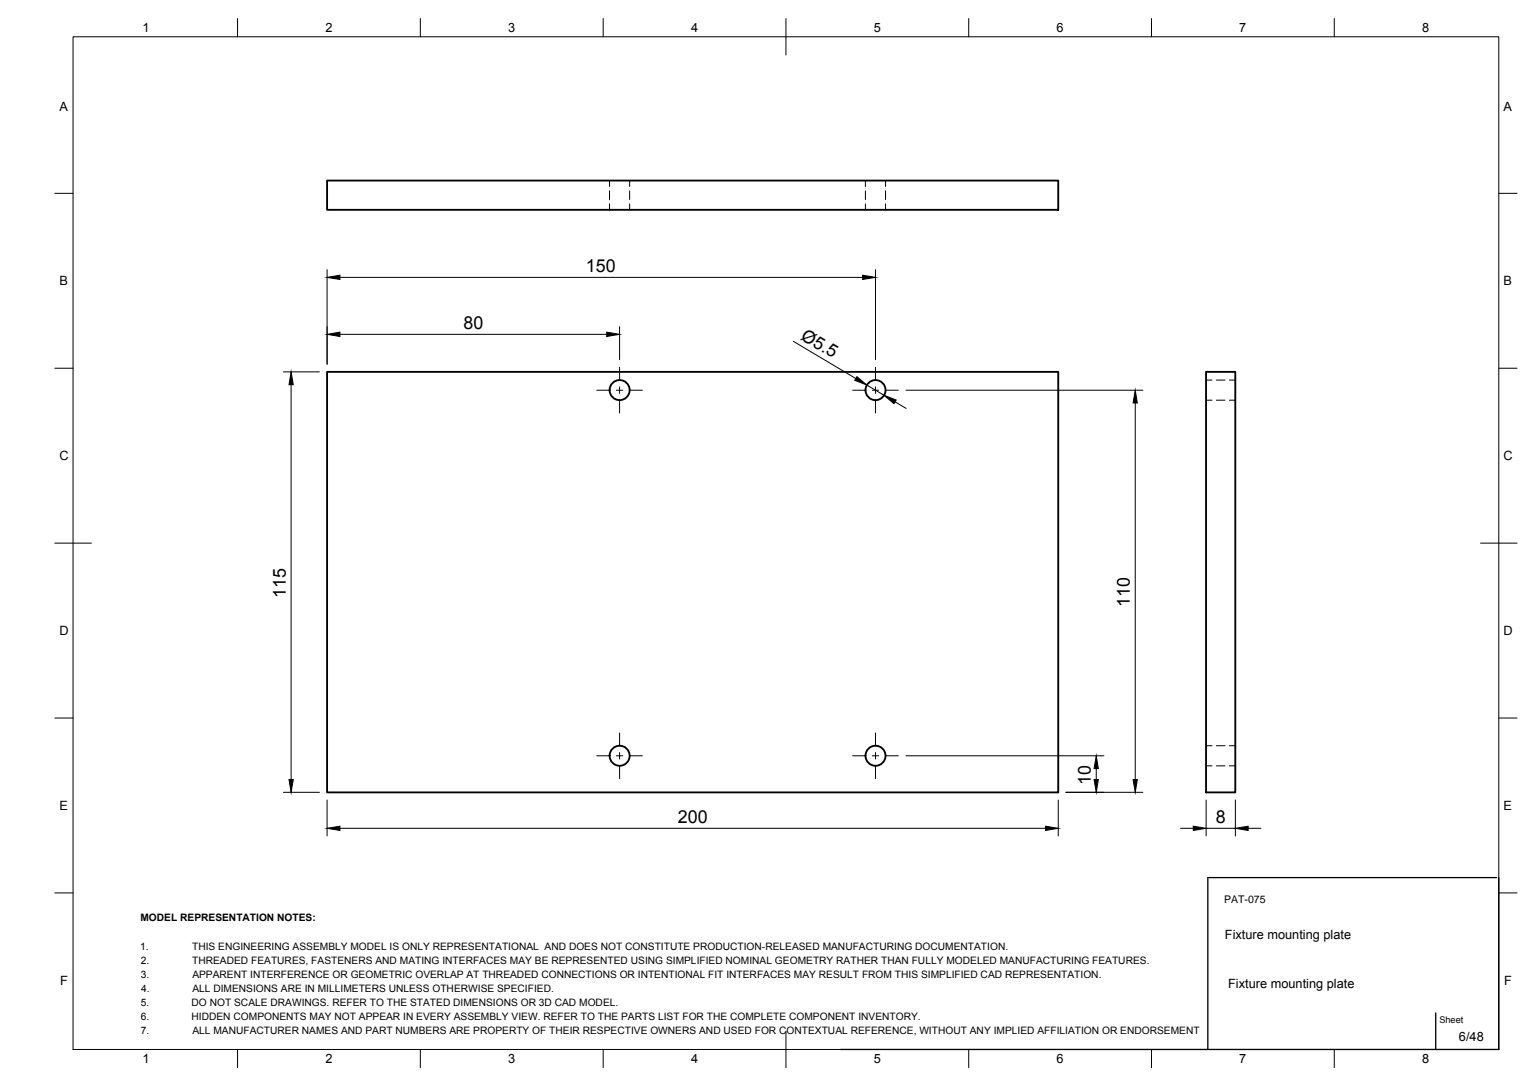
ISO-10303-21;
HEADER;
/* Generated by software containing ST-Developer
 * from STEP Tools, Inc. (www.steptools.com) 
 */

FILE_DESCRIPTION(
/* description */ ('Over-Centre Plunger Toggle Clamp on Slotted Fixture Frame'),
/* implementation_level */ '2;1');

FILE_NAME(
/* name */ 
'Fixture mounting plate.step',
/* time_stamp */ '2026-10-28T03:23:24-07:00',
/* author */ (''),
/* organization */ (''),
/* preprocessor_version */ 'ST-DEVELOPER v20.2',
/* originating_system */ 'Autodesk Translation Framework v15.17.0.0',
/* authorisation */ '');

FILE_SCHEMA (('AUTOMOTIVE_DESIGN { 1 0 10303 214 3 1 1 }'));
ENDSEC;

DATA;
#10=MECHANICAL_DESIGN_GEOMETRIC_PRESENTATION_REPRESENTATION('',(#514),#15212);
#430=SHAPE_REPRESENTATION_RELATIONSHIP('SRR','None',#15404,#472);
#472=ADVANCED_BREP_SHAPE_REPRESENTATION('',(#565),#15166);
#514=STYLED_ITEM('',(#15712),#565);
#565=MANIFOLD_SOLID_BREP('Body1',#8246);
#635=FACE_BOUND('',#1624,.T.);
#636=FACE_BOUND('',#1625,.T.);
#637=FACE_BOUND('',#1626,.T.);
#638=FACE_BOUND('',#1627,.T.);
#639=FACE_BOUND('',#1629,.T.);
#640=FACE_BOUND('',#1630,.T.);
#641=FACE_BOUND('',#1631,.T.);
#642=FACE_BOUND('',#1632,.T.);
#789=PLANE('',#8821);
#790=PLANE('',#8822);
#791=PLANE('',#8823);
#792=PLANE('',#8824);
#793=PLANE('',#8825);
#794=PLANE('',#8826);
#1105=FACE_OUTER_BOUND('',#1615,.T.);
#1106=FACE_OUTER_BOUND('',#1616,.T.);
#1107=FACE_OUTER_BOUND('',#1617,.T.);
#1108=FACE_OUTER_BOUND('',#1618,.T.);
#1109=FACE_OUTER_BOUND('',#1619,.T.);
#1110=FACE_OUTER_BOUND('',#1620,.T.);
#1111=FACE_OUTER_BOUND('',#1621,.T.);
#1112=FACE_OUTER_BOUND('',#1622,.T.);
#1113=FACE_OUTER_BOUND('',#1623,.T.);
#1114=FACE_OUTER_BOUND('',#1628,.T.);
#1615=EDGE_LOOP('',(#5665,#5666,#5667,#5668));
#1616=EDGE_LOOP('',(#5669,#5670,#5671,#5672));
#1617=EDGE_LOOP('',(#5673,#5674,#5675,#5676));
#1618=EDGE_LOOP('',(#5677,#5678,#5679,#5680));
#1619=EDGE_LOOP('',(#5681,#5682,#5683,#5684));
#1620=EDGE_LOOP('',(#5685,#5686,#5687,#5688));
#1621=EDGE_LOOP('',(#5689,#5690,#5691,#5692));
#1622=EDGE_LOOP('',(#5693,#5694,#5695,#5696));
#1623=EDGE_LOOP('',(#5697,#5698,#5699,#5700));
#1624=EDGE_LOOP('',(#5701));
#1625=EDGE_LOOP('',(#5702));
#1626=EDGE_LOOP('',(#5703));
#1627=EDGE_LOOP('',(#5704));
#1628=EDGE_LOOP('',(#5705,#5706,#5707,#5708));
#1629=EDGE_LOOP('',(#5709));
#1630=EDGE_LOOP('',(#5710));
#1631=EDGE_LOOP('',(#5711));
#1632=EDGE_LOOP('',(#5712));
#2255=LINE('',#12472,#2885);
#2256=LINE('',#12478,#2886);
#2257=LINE('',#12484,#2887);
#2258=LINE('',#12490,#2888);
#2259=LINE('',#12495,#2889);
#2260=LINE('',#12497,#2890);
#2261=LINE('',#12499,#2891);
#2262=LINE('',#12500,#2892);
#2263=LINE('',#12503,#2893);
#2264=LINE('',#12505,#2894);
#2265=LINE('',#12506,#2895);
#2266=LINE('',#12509,#2896);
#2267=LINE('',#12511,#2897);
#2268=LINE('',#12512,#2898);
#2269=LINE('',#12514,#2899);
#2270=LINE('',#12515,#2900);
#2885=VECTOR('',#9874,0.275);
#2886=VECTOR('',#9881,0.275);
#2887=VECTOR('',#9888,0.275);
#2888=VECTOR('',#9895,0.275);
#2889=VECTOR('',#9900,1.);
#2890=VECTOR('',#9901,1.);
#2891=VECTOR('',#9902,1.);
#2892=VECTOR('',#9903,1.);
#2893=VECTOR('',#9906,1.);
#2894=VECTOR('',#9907,1.);
#2895=VECTOR('',#9908,1.);
#2896=VECTOR('',#9911,1.);
#2897=VECTOR('',#9912,1.);
#2898=VECTOR('',#9913,1.);
#2899=VECTOR('',#9916,1.);
#2900=VECTOR('',#9917,1.);
#3515=CIRCLE('',#8810,0.275);
#3516=CIRCLE('',#8811,0.275);
#3517=CIRCLE('',#8813,0.275);
#3518=CIRCLE('',#8814,0.275);
#3519=CIRCLE('',#8816,0.275);
#3520=CIRCLE('',#8817,0.275);
#3521=CIRCLE('',#8819,0.275);
#3522=CIRCLE('',#8820,0.275);
#3891=VERTEX_POINT('',#12469);
#3892=VERTEX_POINT('',#12471);
#3893=VERTEX_POINT('',#12475);
#3894=VERTEX_POINT('',#12477);
#3895=VERTEX_POINT('',#12481);
#3896=VERTEX_POINT('',#12483);
#3897=VERTEX_POINT('',#12487);
#3898=VERTEX_POINT('',#12489);
#3899=VERTEX_POINT('',#12493);
#3900=VERTEX_POINT('',#12494);
#3901=VERTEX_POINT('',#12496);
#3902=VERTEX_POINT('',#12498);
#3903=VERTEX_POINT('',#12502);
#3904=VERTEX_POINT('',#12504);
#3905=VERTEX_POINT('',#12508);
#3906=VERTEX_POINT('',#12510);
#4593=EDGE_CURVE('',#3891,#3891,#3515,.T.);
#4594=EDGE_CURVE('',#3891,#3892,#2255,.T.);
#4595=EDGE_CURVE('',#3892,#3892,#3516,.T.);
#4596=EDGE_CURVE('',#3893,#3893,#3517,.T.);
#4597=EDGE_CURVE('',#3893,#3894,#2256,.T.);
#4598=EDGE_CURVE('',#3894,#3894,#3518,.T.);
#4599=EDGE_CURVE('',#3895,#3895,#3519,.T.);
#4600=EDGE_CURVE('',#3895,#3896,#2257,.T.);
#4601=EDGE_CURVE('',#3896,#3896,#3520,.T.);
#4602=EDGE_CURVE('',#3897,#3897,#3521,.T.);
#4603=EDGE_CURVE('',#3897,#3898,#2258,.T.);
#4604=EDGE_CURVE('',#3898,#3898,#3522,.T.);
#4605=EDGE_CURVE('',#3899,#3900,#2259,.T.);
#4606=EDGE_CURVE('',#3900,#3901,#2260,.T.);
#4607=EDGE_CURVE('',#3902,#3901,#2261,.T.);
#4608=EDGE_CURVE('',#3899,#3902,#2262,.T.);
#4609=EDGE_CURVE('',#3903,#3899,#2263,.T.);
#4610=EDGE_CURVE('',#3904,#3902,#2264,.T.);
#4611=EDGE_CURVE('',#3903,#3904,#2265,.T.);
#4612=EDGE_CURVE('',#3905,#3903,#2266,.T.);
#4613=EDGE_CURVE('',#3906,#3904,#2267,.T.);
#4614=EDGE_CURVE('',#3905,#3906,#2268,.T.);
#4615=EDGE_CURVE('',#3900,#3905,#2269,.T.);
#4616=EDGE_CURVE('',#3901,#3906,#2270,.T.);
#5665=ORIENTED_EDGE('',*,*,#4593,.F.);
#5666=ORIENTED_EDGE('',*,*,#4594,.T.);
#5667=ORIENTED_EDGE('',*,*,#4595,.F.);
#5668=ORIENTED_EDGE('',*,*,#4594,.F.);
#5669=ORIENTED_EDGE('',*,*,#4596,.F.);
#5670=ORIENTED_EDGE('',*,*,#4597,.T.);
#5671=ORIENTED_EDGE('',*,*,#4598,.F.);
#5672=ORIENTED_EDGE('',*,*,#4597,.F.);
#5673=ORIENTED_EDGE('',*,*,#4599,.F.);
#5674=ORIENTED_EDGE('',*,*,#4600,.T.);
#5675=ORIENTED_EDGE('',*,*,#4601,.F.);
#5676=ORIENTED_EDGE('',*,*,#4600,.F.);
#5677=ORIENTED_EDGE('',*,*,#4602,.F.);
#5678=ORIENTED_EDGE('',*,*,#4603,.T.);
#5679=ORIENTED_EDGE('',*,*,#4604,.F.);
#5680=ORIENTED_EDGE('',*,*,#4603,.F.);
#5681=ORIENTED_EDGE('',*,*,#4605,.T.);
#5682=ORIENTED_EDGE('',*,*,#4606,.T.);
#5683=ORIENTED_EDGE('',*,*,#4607,.F.);
#5684=ORIENTED_EDGE('',*,*,#4608,.F.);
#5685=ORIENTED_EDGE('',*,*,#4609,.T.);
#5686=ORIENTED_EDGE('',*,*,#4608,.T.);
#5687=ORIENTED_EDGE('',*,*,#4610,.F.);
#5688=ORIENTED_EDGE('',*,*,#4611,.F.);
#5689=ORIENTED_EDGE('',*,*,#4612,.T.);
#5690=ORIENTED_EDGE('',*,*,#4611,.T.);
#5691=ORIENTED_EDGE('',*,*,#4613,.F.);
#5692=ORIENTED_EDGE('',*,*,#4614,.F.);
#5693=ORIENTED_EDGE('',*,*,#4615,.T.);
#5694=ORIENTED_EDGE('',*,*,#4614,.T.);
#5695=ORIENTED_EDGE('',*,*,#4616,.F.);
#5696=ORIENTED_EDGE('',*,*,#4606,.F.);
#5697=ORIENTED_EDGE('',*,*,#4616,.T.);
#5698=ORIENTED_EDGE('',*,*,#4613,.T.);
#5699=ORIENTED_EDGE('',*,*,#4610,.T.);
#5700=ORIENTED_EDGE('',*,*,#4607,.T.);
#5701=ORIENTED_EDGE('',*,*,#4595,.T.);
#5702=ORIENTED_EDGE('',*,*,#4598,.T.);
#5703=ORIENTED_EDGE('',*,*,#4601,.T.);
#5704=ORIENTED_EDGE('',*,*,#4604,.T.);
#5705=ORIENTED_EDGE('',*,*,#4615,.F.);
#5706=ORIENTED_EDGE('',*,*,#4605,.F.);
#5707=ORIENTED_EDGE('',*,*,#4609,.F.);
#5708=ORIENTED_EDGE('',*,*,#4612,.F.);
#5709=ORIENTED_EDGE('',*,*,#4593,.T.);
#5710=ORIENTED_EDGE('',*,*,#4596,.T.);
#5711=ORIENTED_EDGE('',*,*,#4599,.T.);
#5712=ORIENTED_EDGE('',*,*,#4602,.T.);
#7629=CYLINDRICAL_SURFACE('',#8809,0.275);
#7630=CYLINDRICAL_SURFACE('',#8812,0.275);
#7631=CYLINDRICAL_SURFACE('',#8815,0.275);
#7632=CYLINDRICAL_SURFACE('',#8818,0.275);
#7777=ADVANCED_FACE('',(#1105),#7629,.F.);
#7778=ADVANCED_FACE('',(#1106),#7630,.F.);
#7779=ADVANCED_FACE('',(#1107),#7631,.F.);
#7780=ADVANCED_FACE('',(#1108),#7632,.F.);
#7781=ADVANCED_FACE('',(#1109),#789,.T.);
#7782=ADVANCED_FACE('',(#1110),#790,.T.);
#7783=ADVANCED_FACE('',(#1111),#791,.T.);
#7784=ADVANCED_FACE('',(#1112),#792,.T.);
#7785=ADVANCED_FACE('',(#1113,#635,#636,#637,#638),#793,.T.);
#7786=ADVANCED_FACE('',(#1114,#639,#640,#641,#642),#794,.F.);
#8246=CLOSED_SHELL('',(#7777,#7778,#7779,#7780,#7781,#7782,#7783,#7784,
#7785,#7786));
#8808=AXIS2_PLACEMENT_3D('',#12467,#9868,#9869);
#8809=AXIS2_PLACEMENT_3D('',#12468,#9870,#9871);
#8810=AXIS2_PLACEMENT_3D('',#12470,#9872,#9873);
#8811=AXIS2_PLACEMENT_3D('',#12473,#9875,#9876);
#8812=AXIS2_PLACEMENT_3D('',#12474,#9877,#9878);
#8813=AXIS2_PLACEMENT_3D('',#12476,#9879,#9880);
#8814=AXIS2_PLACEMENT_3D('',#12479,#9882,#9883);
#8815=AXIS2_PLACEMENT_3D('',#12480,#9884,#9885);
#8816=AXIS2_PLACEMENT_3D('',#12482,#9886,#9887);
#8817=AXIS2_PLACEMENT_3D('',#12485,#9889,#9890);
#8818=AXIS2_PLACEMENT_3D('',#12486,#9891,#9892);
#8819=AXIS2_PLACEMENT_3D('',#12488,#9893,#9894);
#8820=AXIS2_PLACEMENT_3D('',#12491,#9896,#9897);
#8821=AXIS2_PLACEMENT_3D('',#12492,#9898,#9899);
#8822=AXIS2_PLACEMENT_3D('',#12501,#9904,#9905);
#8823=AXIS2_PLACEMENT_3D('',#12507,#9909,#9910);
#8824=AXIS2_PLACEMENT_3D('',#12513,#9914,#9915);
#8825=AXIS2_PLACEMENT_3D('',#12516,#9918,#9919);
#8826=AXIS2_PLACEMENT_3D('',#12517,#9920,#9921);
#9868=DIRECTION('axis',(0.,0.,1.));
#9869=DIRECTION('refdir',(1.,0.,0.));
#9870=DIRECTION('center_axis',(0.,0.,1.));
#9871=DIRECTION('ref_axis',(1.,0.,0.));
#9872=DIRECTION('center_axis',(0.,0.,1.));
#9873=DIRECTION('ref_axis',(1.,0.,0.));
#9874=DIRECTION('',(0.,0.,1.));
#9875=DIRECTION('center_axis',(0.,0.,-1.));
#9876=DIRECTION('ref_axis',(1.,0.,0.));
#9877=DIRECTION('center_axis',(0.,0.,1.));
#9878=DIRECTION('ref_axis',(1.,0.,0.));
#9879=DIRECTION('center_axis',(0.,0.,1.));
#9880=DIRECTION('ref_axis',(1.,0.,0.));
#9881=DIRECTION('',(0.,0.,1.));
#9882=DIRECTION('center_axis',(0.,0.,-1.));
#9883=DIRECTION('ref_axis',(1.,0.,0.));
#9884=DIRECTION('center_axis',(0.,0.,1.));
#9885=DIRECTION('ref_axis',(1.,0.,0.));
#9886=DIRECTION('center_axis',(0.,0.,1.));
#9887=DIRECTION('ref_axis',(1.,0.,0.));
#9888=DIRECTION('',(0.,0.,1.));
#9889=DIRECTION('center_axis',(0.,0.,-1.));
#9890=DIRECTION('ref_axis',(1.,0.,0.));
#9891=DIRECTION('center_axis',(0.,0.,1.));
#9892=DIRECTION('ref_axis',(1.,0.,0.));
#9893=DIRECTION('center_axis',(0.,0.,1.));
#9894=DIRECTION('ref_axis',(1.,0.,0.));
#9895=DIRECTION('',(0.,0.,1.));
#9896=DIRECTION('center_axis',(0.,0.,-1.));
#9897=DIRECTION('ref_axis',(1.,0.,0.));
#9898=DIRECTION('center_axis',(0.,1.,0.));
#9899=DIRECTION('ref_axis',(-1.,0.,0.));
#9900=DIRECTION('',(-1.,0.,0.));
#9901=DIRECTION('',(0.,0.,1.));
#9902=DIRECTION('',(-1.,0.,0.));
#9903=DIRECTION('',(0.,0.,1.));
#9904=DIRECTION('center_axis',(1.,0.,0.));
#9905=DIRECTION('ref_axis',(0.,1.,0.));
#9906=DIRECTION('',(0.,1.,0.));
#9907=DIRECTION('',(0.,1.,0.));
#9908=DIRECTION('',(0.,0.,1.));
#9909=DIRECTION('center_axis',(0.,-1.,0.));
#9910=DIRECTION('ref_axis',(1.,0.,0.));
#9911=DIRECTION('',(1.,0.,0.));
#9912=DIRECTION('',(1.,0.,0.));
#9913=DIRECTION('',(0.,0.,1.));
#9914=DIRECTION('center_axis',(-1.,0.,0.));
#9915=DIRECTION('ref_axis',(0.,-1.,0.));
#9916=DIRECTION('',(0.,-1.,0.));
#9917=DIRECTION('',(0.,-1.,0.));
#9918=DIRECTION('center_axis',(0.,0.,1.));
#9919=DIRECTION('ref_axis',(1.,0.,0.));
#9920=DIRECTION('center_axis',(0.,0.,1.));
#9921=DIRECTION('ref_axis',(1.,0.,0.));
#12467=CARTESIAN_POINT('',(0.,0.,0.));
#12468=CARTESIAN_POINT('Origin',(2.5,4.,-2.9));
#12469=CARTESIAN_POINT('',(2.225,4.,-2.8));
#12470=CARTESIAN_POINT('Origin',(2.5,4.,-2.8));
#12471=CARTESIAN_POINT('',(2.225,4.,-2.));
#12472=CARTESIAN_POINT('',(2.225,4.,-2.9));
#12473=CARTESIAN_POINT('Origin',(2.5,4.,-2.));
#12474=CARTESIAN_POINT('Origin',(-4.5,4.,-2.9));
#12475=CARTESIAN_POINT('',(-4.775,4.,-2.8));
#12476=CARTESIAN_POINT('Origin',(-4.5,4.,-2.8));
#12477=CARTESIAN_POINT('',(-4.775,4.,-2.));
#12478=CARTESIAN_POINT('',(-4.775,4.,-2.9));
#12479=CARTESIAN_POINT('Origin',(-4.5,4.,-2.));
#12480=CARTESIAN_POINT('Origin',(2.5,-6.,-2.9));
#12481=CARTESIAN_POINT('',(2.225,-6.,-2.8));
#12482=CARTESIAN_POINT('Origin',(2.5,-6.,-2.8));
#12483=CARTESIAN_POINT('',(2.225,-6.,-2.));
#12484=CARTESIAN_POINT('',(2.225,-6.,-2.9));
#12485=CARTESIAN_POINT('Origin',(2.5,-6.,-2.));
#12486=CARTESIAN_POINT('Origin',(-4.5,-6.,-2.9));
#12487=CARTESIAN_POINT('',(-4.775,-6.,-2.8));
#12488=CARTESIAN_POINT('Origin',(-4.5,-6.,-2.8));
#12489=CARTESIAN_POINT('',(-4.775,-6.,-2.));
#12490=CARTESIAN_POINT('',(-4.775,-6.,-2.9));
#12491=CARTESIAN_POINT('Origin',(-4.5,-6.,-2.));
#12492=CARTESIAN_POINT('Origin',(10.5,4.5,-2.8));
#12493=CARTESIAN_POINT('',(10.5,4.5,-2.8));
#12494=CARTESIAN_POINT('',(-9.5,4.5,-2.8));
#12495=CARTESIAN_POINT('',(10.5,4.5,-2.8));
#12496=CARTESIAN_POINT('',(-9.5,4.5,-2.));
#12497=CARTESIAN_POINT('',(-9.5,4.5,-2.8));
#12498=CARTESIAN_POINT('',(10.5,4.5,-2.));
#12499=CARTESIAN_POINT('',(10.5,4.5,-2.));
#12500=CARTESIAN_POINT('',(10.5,4.5,-2.8));
#12501=CARTESIAN_POINT('Origin',(10.5,-7.,-2.8));
#12502=CARTESIAN_POINT('',(10.5,-7.,-2.8));
#12503=CARTESIAN_POINT('',(10.5,-7.,-2.8));
#12504=CARTESIAN_POINT('',(10.5,-7.,-2.));
#12505=CARTESIAN_POINT('',(10.5,-7.,-2.));
#12506=CARTESIAN_POINT('',(10.5,-7.,-2.8));
#12507=CARTESIAN_POINT('Origin',(-9.5,-7.,-2.8));
#12508=CARTESIAN_POINT('',(-9.5,-7.,-2.8));
#12509=CARTESIAN_POINT('',(-9.5,-7.,-2.8));
#12510=CARTESIAN_POINT('',(-9.5,-7.,-2.));
#12511=CARTESIAN_POINT('',(-9.5,-7.,-2.));
#12512=CARTESIAN_POINT('',(-9.5,-7.,-2.8));
#12513=CARTESIAN_POINT('Origin',(-9.5,4.5,-2.8));
#12514=CARTESIAN_POINT('',(-9.5,4.5,-2.8));
#12515=CARTESIAN_POINT('',(-9.5,4.5,-2.));
#12516=CARTESIAN_POINT('Origin',(0.5,-1.25,-2.));
#12517=CARTESIAN_POINT('Origin',(0.5,-1.25,-2.8));
#15116=UNCERTAINTY_MEASURE_WITH_UNIT(LENGTH_MEASURE(0.001),#15213,
'DISTANCE_ACCURACY_VALUE',
'Maximum model space distance between geometric entities at asserted c
onnectivities');
#15162=UNCERTAINTY_MEASURE_WITH_UNIT(LENGTH_MEASURE(0.001),#15213,
'DISTANCE_ACCURACY_VALUE',
'Maximum model space distance between geometric entities at asserted c
onnectivities');
#15166=(
GEOMETRIC_REPRESENTATION_CONTEXT(3)
GLOBAL_UNCERTAINTY_ASSIGNED_CONTEXT((#15116))
GLOBAL_UNIT_ASSIGNED_CONTEXT((#15213,#15215,#15216))
REPRESENTATION_CONTEXT('','3D')
);
#15212=(
GEOMETRIC_REPRESENTATION_CONTEXT(3)
GLOBAL_UNCERTAINTY_ASSIGNED_CONTEXT((#15162))
GLOBAL_UNIT_ASSIGNED_CONTEXT((#15213,#15215,#15216))
REPRESENTATION_CONTEXT('','3D')
);
#15213=(
LENGTH_UNIT()
NAMED_UNIT(*)
SI_UNIT(.CENTI.,.METRE.)
);
#15215=(
NAMED_UNIT(*)
PLANE_ANGLE_UNIT()
SI_UNIT($,.RADIAN.)
);
#15216=(
NAMED_UNIT(*)
SI_UNIT($,.STERADIAN.)
SOLID_ANGLE_UNIT()
);
#15220=SHAPE_DEFINITION_REPRESENTATION(#15269,#15404);
#15269=PRODUCT_DEFINITION_SHAPE('',$,#15454);
#15404=SHAPE_REPRESENTATION('',(#8808),#15166);
#15450=PRODUCT_DEFINITION_CONTEXT('part definition',#15599,'design');
#15454=PRODUCT_DEFINITION('Fixture mounting plate',
'Fixture mounting plate',#15503,#15450);
#15503=PRODUCT_DEFINITION_FORMATION('',$,#15604);
#15599=APPLICATION_CONTEXT(
'Core Data for Automotive Mechanical Design Process');
#15600=PRODUCT_CONTEXT('part definition',#15599,'mechanical');
#15604=PRODUCT('Fixture mounting plate','Fixture mounting plate',
'Fixture mounting plate',(#15600));
#15706=COLOUR_RGB('Sky Blue',0.24,0.69,0.87);
#15707=FILL_AREA_STYLE_COLOUR('',#15706);
#15708=FILL_AREA_STYLE('',(#15707));
#15709=SURFACE_STYLE_FILL_AREA(#15708);
#15710=SURFACE_SIDE_STYLE('',(#15709));
#15711=SURFACE_STYLE_USAGE(.BOTH.,#15710);
#15712=PRESENTATION_STYLE_ASSIGNMENT((#15711));
ENDSEC;
END-ISO-10303-21;
